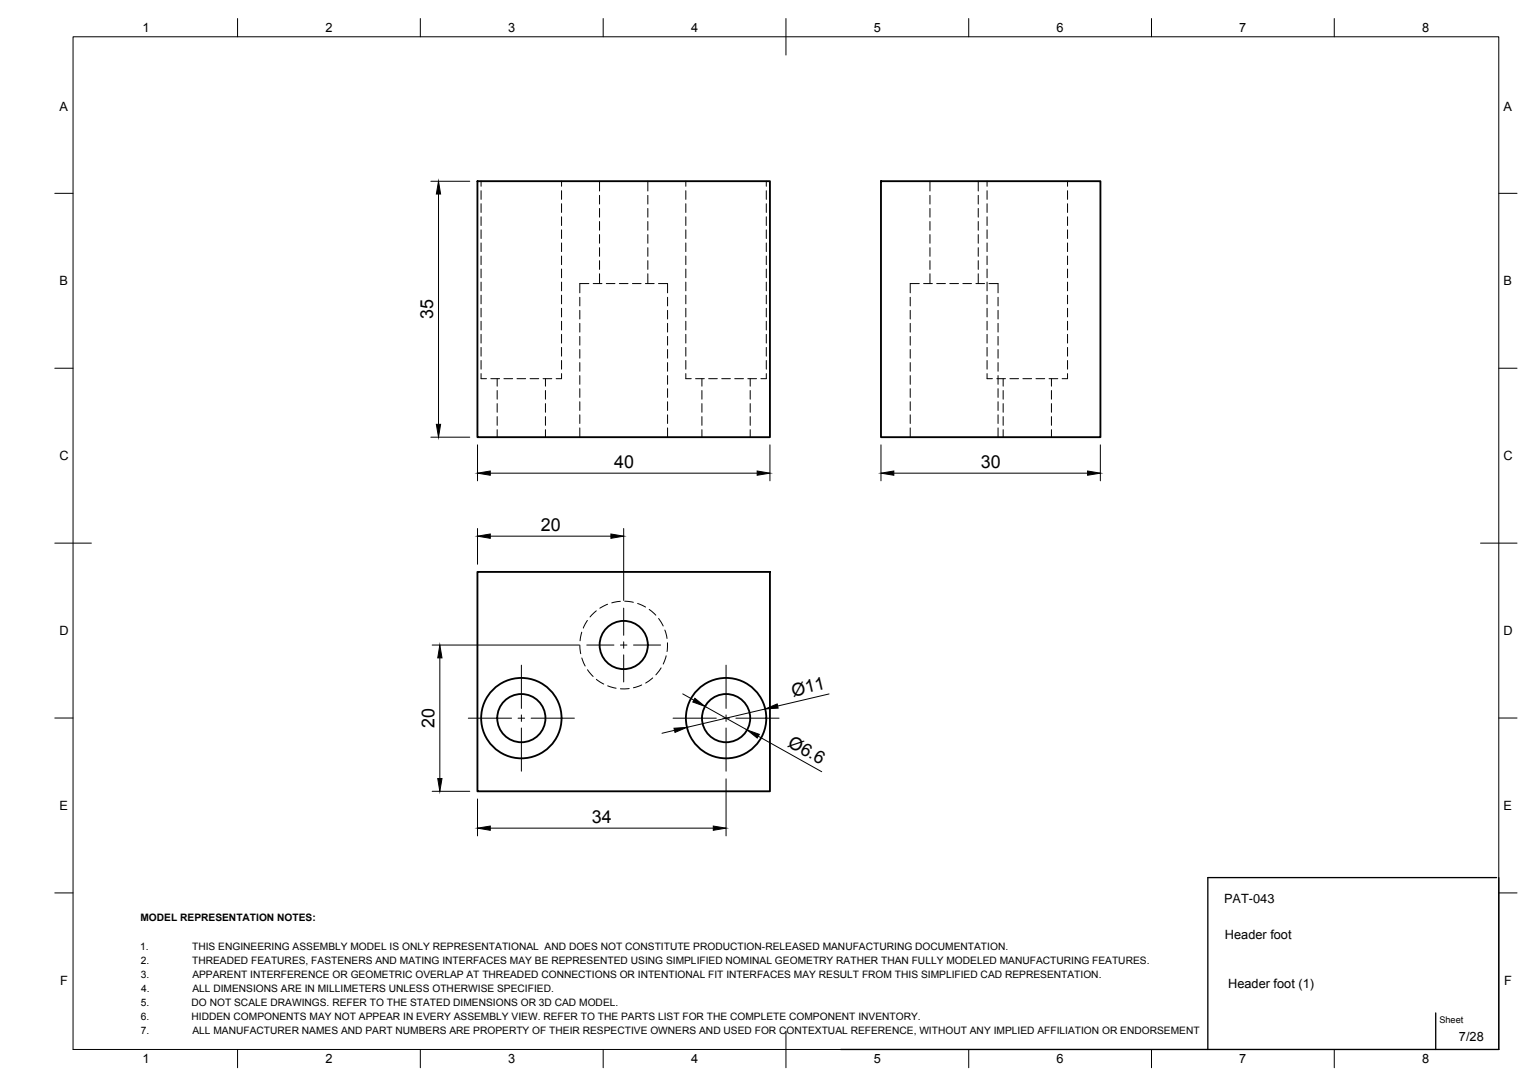
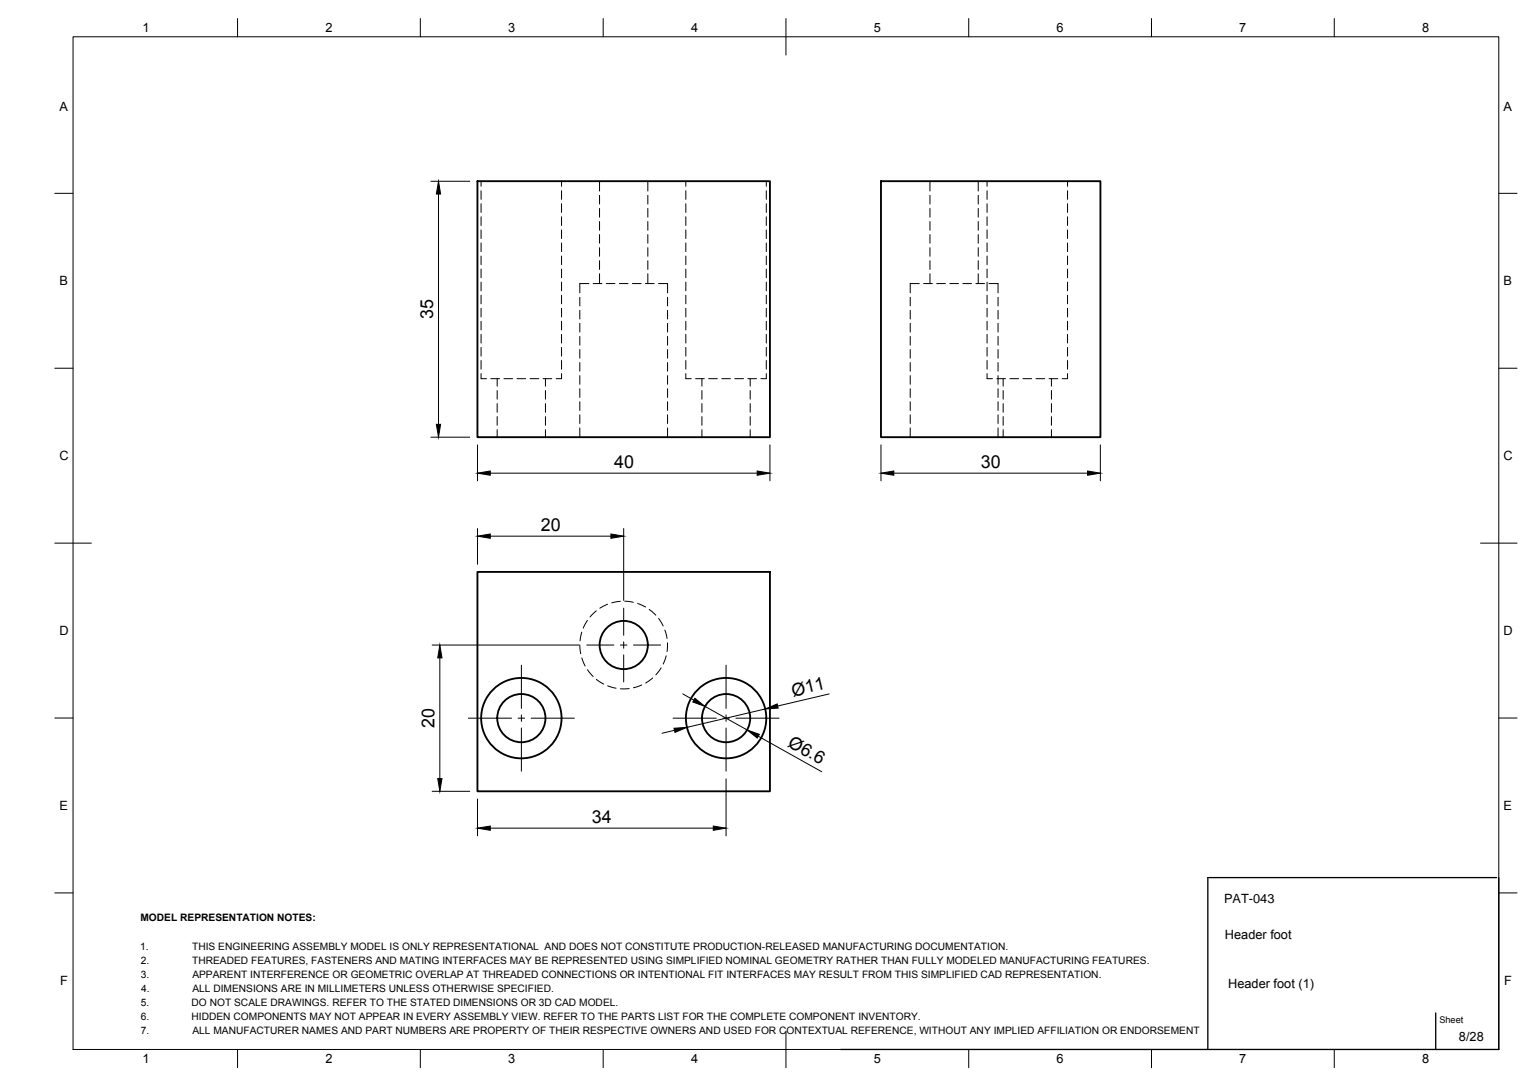
ISO-10303-21;
HEADER;
/* Generated by software containing ST-Developer
 * from STEP Tools, Inc. (www.steptools.com) 
 */

FILE_DESCRIPTION(
/* description */ ('Four-valve pipe header'),
/* implementation_level */ '2;1');

FILE_NAME(
/* name */ 'Header foot.step',
/* time_stamp */ '2026-10-29T16:56:19-07:00',
/* author */ (''),
/* organization */ (''),
/* preprocessor_version */ 'ST-DEVELOPER v20.2',
/* originating_system */ 'Autodesk Translation Framework v15.17.0.0',
/* authorisation */ '');

FILE_SCHEMA (('AUTOMOTIVE_DESIGN { 1 0 10303 214 3 1 1 }'));
ENDSEC;

DATA;
#10=MECHANICAL_DESIGN_GEOMETRIC_PRESENTATION_REPRESENTATION('',(#335),#10119);
#283=SHAPE_REPRESENTATION_RELATIONSHIP('SRR','None',#10244,#309);
#309=ADVANCED_BREP_SHAPE_REPRESENTATION('',(#361),#10093);
#335=STYLED_ITEM('',(#10463),#361);
#361=MANIFOLD_SOLID_BREP('Body1',#5581);
#437=FACE_BOUND('',#1153,.T.);
#438=FACE_BOUND('',#1157,.T.);
#439=FACE_BOUND('',#1161,.T.);
#440=FACE_BOUND('',#1168,.T.);
#441=FACE_BOUND('',#1169,.T.);
#442=FACE_BOUND('',#1170,.T.);
#443=FACE_BOUND('',#1172,.T.);
#444=FACE_BOUND('',#1173,.T.);
#445=FACE_BOUND('',#1174,.T.);
#570=PLANE('',#6036);
#571=PLANE('',#6043);
#572=PLANE('',#6050);
#573=PLANE('',#6054);
#574=PLANE('',#6055);
#575=PLANE('',#6056);
#576=PLANE('',#6057);
#577=PLANE('',#6058);
#578=PLANE('',#6059);
#808=FACE_OUTER_BOUND('',#1151,.T.);
#809=FACE_OUTER_BOUND('',#1152,.T.);
#810=FACE_OUTER_BOUND('',#1154,.T.);
#811=FACE_OUTER_BOUND('',#1155,.T.);
#812=FACE_OUTER_BOUND('',#1156,.T.);
#813=FACE_OUTER_BOUND('',#1158,.T.);
#814=FACE_OUTER_BOUND('',#1159,.T.);
#815=FACE_OUTER_BOUND('',#1160,.T.);
#816=FACE_OUTER_BOUND('',#1162,.T.);
#817=FACE_OUTER_BOUND('',#1163,.T.);
#818=FACE_OUTER_BOUND('',#1164,.T.);
#819=FACE_OUTER_BOUND('',#1165,.T.);
#820=FACE_OUTER_BOUND('',#1166,.T.);
#821=FACE_OUTER_BOUND('',#1167,.T.);
#822=FACE_OUTER_BOUND('',#1171,.T.);
#1151=EDGE_LOOP('',(#4045,#4046,#4047,#4048));
#1152=EDGE_LOOP('',(#4049));
#1153=EDGE_LOOP('',(#4050));
#1154=EDGE_LOOP('',(#4051,#4052,#4053,#4054));
#1155=EDGE_LOOP('',(#4055,#4056,#4057,#4058));
#1156=EDGE_LOOP('',(#4059));
#1157=EDGE_LOOP('',(#4060));
#1158=EDGE_LOOP('',(#4061,#4062,#4063,#4064));
#1159=EDGE_LOOP('',(#4065,#4066,#4067,#4068));
#1160=EDGE_LOOP('',(#4069));
#1161=EDGE_LOOP('',(#4070));
#1162=EDGE_LOOP('',(#4071,#4072,#4073,#4074));
#1163=EDGE_LOOP('',(#4075,#4076,#4077,#4078));
#1164=EDGE_LOOP('',(#4079,#4080,#4081,#4082));
#1165=EDGE_LOOP('',(#4083,#4084,#4085,#4086));
#1166=EDGE_LOOP('',(#4087,#4088,#4089,#4090));
#1167=EDGE_LOOP('',(#4091,#4092,#4093,#4094));
#1168=EDGE_LOOP('',(#4095));
#1169=EDGE_LOOP('',(#4096));
#1170=EDGE_LOOP('',(#4097));
#1171=EDGE_LOOP('',(#4098,#4099,#4100,#4101));
#1172=EDGE_LOOP('',(#4102));
#1173=EDGE_LOOP('',(#4103));
#1174=EDGE_LOOP('',(#4104));
#1588=LINE('',#8761,#2006);
#1589=LINE('',#8769,#2007);
#1590=LINE('',#8774,#2008);
#1591=LINE('',#8782,#2009);
#1592=LINE('',#8787,#2010);
#1593=LINE('',#8794,#2011);
#1594=LINE('',#8799,#2012);
#1595=LINE('',#8801,#2013);
#1596=LINE('',#8803,#2014);
#1597=LINE('',#8804,#2015);
#1598=LINE('',#8807,#2016);
#1599=LINE('',#8809,#2017);
#1600=LINE('',#8810,#2018);
#1601=LINE('',#8813,#2019);
#1602=LINE('',#8815,#2020);
#1603=LINE('',#8816,#2021);
#1604=LINE('',#8818,#2022);
#1605=LINE('',#8819,#2023);
#2006=VECTOR('',#6917,0.55);
#2007=VECTOR('',#6928,0.33);
#2008=VECTOR('',#6933,0.55);
#2009=VECTOR('',#6944,0.33);
#2010=VECTOR('',#6949,0.6);
#2011=VECTOR('',#6958,0.33);
#2012=VECTOR('',#6963,1.);
#2013=VECTOR('',#6964,1.);
#2014=VECTOR('',#6965,1.);
#2015=VECTOR('',#6966,1.);
#2016=VECTOR('',#6969,1.);
#2017=VECTOR('',#6970,1.);
#2018=VECTOR('',#6971,1.);
#2019=VECTOR('',#6974,1.);
#2020=VECTOR('',#6975,1.);
#2021=VECTOR('',#6976,1.);
#2022=VECTOR('',#6979,1.);
#2023=VECTOR('',#6980,1.);
#2396=CIRCLE('',#6034,0.55);
#2397=CIRCLE('',#6035,0.55);
#2398=CIRCLE('',#6037,0.33);
#2399=CIRCLE('',#6039,0.33);
#2400=CIRCLE('',#6041,0.55);
#2401=CIRCLE('',#6042,0.55);
#2402=CIRCLE('',#6044,0.33);
#2403=CIRCLE('',#6046,0.33);
#2404=CIRCLE('',#6048,0.6);
#2405=CIRCLE('',#6049,0.6);
#2406=CIRCLE('',#6051,0.33);
#2407=CIRCLE('',#6053,0.33);
#2676=VERTEX_POINT('',#8758);
#2677=VERTEX_POINT('',#8760);
#2678=VERTEX_POINT('',#8764);
#2679=VERTEX_POINT('',#8767);
#2680=VERTEX_POINT('',#8771);
#2681=VERTEX_POINT('',#8773);
#2682=VERTEX_POINT('',#8777);
#2683=VERTEX_POINT('',#8780);
#2684=VERTEX_POINT('',#8784);
#2685=VERTEX_POINT('',#8786);
#2686=VERTEX_POINT('',#8790);
#2687=VERTEX_POINT('',#8793);
#2688=VERTEX_POINT('',#8797);
#2689=VERTEX_POINT('',#8798);
#2690=VERTEX_POINT('',#8800);
#2691=VERTEX_POINT('',#8802);
#2692=VERTEX_POINT('',#8806);
#2693=VERTEX_POINT('',#8808);
#2694=VERTEX_POINT('',#8812);
#2695=VERTEX_POINT('',#8814);
#3189=EDGE_CURVE('',#2676,#2676,#2396,.T.);
#3190=EDGE_CURVE('',#2676,#2677,#1588,.T.);
#3191=EDGE_CURVE('',#2677,#2677,#2397,.T.);
#3192=EDGE_CURVE('',#2678,#2678,#2398,.T.);
#3193=EDGE_CURVE('',#2679,#2679,#2399,.T.);
#3194=EDGE_CURVE('',#2679,#2678,#1589,.T.);
#3195=EDGE_CURVE('',#2680,#2680,#2400,.T.);
#3196=EDGE_CURVE('',#2680,#2681,#1590,.T.);
#3197=EDGE_CURVE('',#2681,#2681,#2401,.T.);
#3198=EDGE_CURVE('',#2682,#2682,#2402,.T.);
#3199=EDGE_CURVE('',#2683,#2683,#2403,.T.);
#3200=EDGE_CURVE('',#2683,#2682,#1591,.T.);
#3201=EDGE_CURVE('',#2684,#2684,#2404,.T.);
#3202=EDGE_CURVE('',#2684,#2685,#1592,.T.);
#3203=EDGE_CURVE('',#2685,#2685,#2405,.T.);
#3204=EDGE_CURVE('',#2686,#2686,#2406,.T.);
#3205=EDGE_CURVE('',#2686,#2687,#1593,.T.);
#3206=EDGE_CURVE('',#2687,#2687,#2407,.T.);
#3207=EDGE_CURVE('',#2688,#2689,#1594,.T.);
#3208=EDGE_CURVE('',#2689,#2690,#1595,.T.);
#3209=EDGE_CURVE('',#2691,#2690,#1596,.T.);
#3210=EDGE_CURVE('',#2688,#2691,#1597,.T.);
#3211=EDGE_CURVE('',#2692,#2688,#1598,.T.);
#3212=EDGE_CURVE('',#2693,#2691,#1599,.T.);
#3213=EDGE_CURVE('',#2692,#2693,#1600,.T.);
#3214=EDGE_CURVE('',#2694,#2692,#1601,.T.);
#3215=EDGE_CURVE('',#2695,#2693,#1602,.T.);
#3216=EDGE_CURVE('',#2694,#2695,#1603,.T.);
#3217=EDGE_CURVE('',#2689,#2694,#1604,.T.);
#3218=EDGE_CURVE('',#2690,#2695,#1605,.T.);
#4045=ORIENTED_EDGE('',*,*,#3189,.F.);
#4046=ORIENTED_EDGE('',*,*,#3190,.T.);
#4047=ORIENTED_EDGE('',*,*,#3191,.F.);
#4048=ORIENTED_EDGE('',*,*,#3190,.F.);
#4049=ORIENTED_EDGE('',*,*,#3189,.T.);
#4050=ORIENTED_EDGE('',*,*,#3192,.F.);
#4051=ORIENTED_EDGE('',*,*,#3193,.F.);
#4052=ORIENTED_EDGE('',*,*,#3194,.T.);
#4053=ORIENTED_EDGE('',*,*,#3192,.T.);
#4054=ORIENTED_EDGE('',*,*,#3194,.F.);
#4055=ORIENTED_EDGE('',*,*,#3195,.F.);
#4056=ORIENTED_EDGE('',*,*,#3196,.T.);
#4057=ORIENTED_EDGE('',*,*,#3197,.F.);
#4058=ORIENTED_EDGE('',*,*,#3196,.F.);
#4059=ORIENTED_EDGE('',*,*,#3195,.T.);
#4060=ORIENTED_EDGE('',*,*,#3198,.F.);
#4061=ORIENTED_EDGE('',*,*,#3199,.F.);
#4062=ORIENTED_EDGE('',*,*,#3200,.T.);
#4063=ORIENTED_EDGE('',*,*,#3198,.T.);
#4064=ORIENTED_EDGE('',*,*,#3200,.F.);
#4065=ORIENTED_EDGE('',*,*,#3201,.F.);
#4066=ORIENTED_EDGE('',*,*,#3202,.T.);
#4067=ORIENTED_EDGE('',*,*,#3203,.T.);
#4068=ORIENTED_EDGE('',*,*,#3202,.F.);
#4069=ORIENTED_EDGE('',*,*,#3203,.F.);
#4070=ORIENTED_EDGE('',*,*,#3204,.F.);
#4071=ORIENTED_EDGE('',*,*,#3204,.T.);
#4072=ORIENTED_EDGE('',*,*,#3205,.T.);
#4073=ORIENTED_EDGE('',*,*,#3206,.F.);
#4074=ORIENTED_EDGE('',*,*,#3205,.F.);
#4075=ORIENTED_EDGE('',*,*,#3207,.T.);
#4076=ORIENTED_EDGE('',*,*,#3208,.T.);
#4077=ORIENTED_EDGE('',*,*,#3209,.F.);
#4078=ORIENTED_EDGE('',*,*,#3210,.F.);
#4079=ORIENTED_EDGE('',*,*,#3211,.T.);
#4080=ORIENTED_EDGE('',*,*,#3210,.T.);
#4081=ORIENTED_EDGE('',*,*,#3212,.F.);
#4082=ORIENTED_EDGE('',*,*,#3213,.F.);
#4083=ORIENTED_EDGE('',*,*,#3214,.T.);
#4084=ORIENTED_EDGE('',*,*,#3213,.T.);
#4085=ORIENTED_EDGE('',*,*,#3215,.F.);
#4086=ORIENTED_EDGE('',*,*,#3216,.F.);
#4087=ORIENTED_EDGE('',*,*,#3217,.T.);
#4088=ORIENTED_EDGE('',*,*,#3216,.T.);
#4089=ORIENTED_EDGE('',*,*,#3218,.F.);
#4090=ORIENTED_EDGE('',*,*,#3208,.F.);
#4091=ORIENTED_EDGE('',*,*,#3218,.T.);
#4092=ORIENTED_EDGE('',*,*,#3215,.T.);
#4093=ORIENTED_EDGE('',*,*,#3212,.T.);
#4094=ORIENTED_EDGE('',*,*,#3209,.T.);
#4095=ORIENTED_EDGE('',*,*,#3191,.T.);
#4096=ORIENTED_EDGE('',*,*,#3197,.T.);
#4097=ORIENTED_EDGE('',*,*,#3206,.T.);
#4098=ORIENTED_EDGE('',*,*,#3217,.F.);
#4099=ORIENTED_EDGE('',*,*,#3207,.F.);
#4100=ORIENTED_EDGE('',*,*,#3211,.F.);
#4101=ORIENTED_EDGE('',*,*,#3214,.F.);
#4102=ORIENTED_EDGE('',*,*,#3193,.T.);
#4103=ORIENTED_EDGE('',*,*,#3199,.T.);
#4104=ORIENTED_EDGE('',*,*,#3201,.T.);
#5175=CYLINDRICAL_SURFACE('',#6033,0.55);
#5176=CYLINDRICAL_SURFACE('',#6038,0.33);
#5177=CYLINDRICAL_SURFACE('',#6040,0.55);
#5178=CYLINDRICAL_SURFACE('',#6045,0.33);
#5179=CYLINDRICAL_SURFACE('',#6047,0.6);
#5180=CYLINDRICAL_SURFACE('',#6052,0.33);
#5308=ADVANCED_FACE('',(#808),#5175,.F.);
#5309=ADVANCED_FACE('',(#809,#437),#570,.T.);
#5310=ADVANCED_FACE('',(#810),#5176,.F.);
#5311=ADVANCED_FACE('',(#811),#5177,.F.);
#5312=ADVANCED_FACE('',(#812,#438),#571,.T.);
#5313=ADVANCED_FACE('',(#813),#5178,.F.);
#5314=ADVANCED_FACE('',(#814),#5179,.F.);
#5315=ADVANCED_FACE('',(#815,#439),#572,.F.);
#5316=ADVANCED_FACE('',(#816),#5180,.F.);
#5317=ADVANCED_FACE('',(#817),#573,.T.);
#5318=ADVANCED_FACE('',(#818),#574,.T.);
#5319=ADVANCED_FACE('',(#819),#575,.T.);
#5320=ADVANCED_FACE('',(#820),#576,.T.);
#5321=ADVANCED_FACE('',(#821,#440,#441,#442),#577,.T.);
#5322=ADVANCED_FACE('',(#822,#443,#444,#445),#578,.F.);
#5581=CLOSED_SHELL('',(#5308,#5309,#5310,#5311,#5312,#5313,#5314,#5315,
#5316,#5317,#5318,#5319,#5320,#5321,#5322));
#6032=AXIS2_PLACEMENT_3D('',#8756,#6911,#6912);
#6033=AXIS2_PLACEMENT_3D('',#8757,#6913,#6914);
#6034=AXIS2_PLACEMENT_3D('',#8759,#6915,#6916);
#6035=AXIS2_PLACEMENT_3D('',#8762,#6918,#6919);
#6036=AXIS2_PLACEMENT_3D('',#8763,#6920,#6921);
#6037=AXIS2_PLACEMENT_3D('',#8765,#6922,#6923);
#6038=AXIS2_PLACEMENT_3D('',#8766,#6924,#6925);
#6039=AXIS2_PLACEMENT_3D('',#8768,#6926,#6927);
#6040=AXIS2_PLACEMENT_3D('',#8770,#6929,#6930);
#6041=AXIS2_PLACEMENT_3D('',#8772,#6931,#6932);
#6042=AXIS2_PLACEMENT_3D('',#8775,#6934,#6935);
#6043=AXIS2_PLACEMENT_3D('',#8776,#6936,#6937);
#6044=AXIS2_PLACEMENT_3D('',#8778,#6938,#6939);
#6045=AXIS2_PLACEMENT_3D('',#8779,#6940,#6941);
#6046=AXIS2_PLACEMENT_3D('',#8781,#6942,#6943);
#6047=AXIS2_PLACEMENT_3D('',#8783,#6945,#6946);
#6048=AXIS2_PLACEMENT_3D('',#8785,#6947,#6948);
#6049=AXIS2_PLACEMENT_3D('',#8788,#6950,#6951);
#6050=AXIS2_PLACEMENT_3D('',#8789,#6952,#6953);
#6051=AXIS2_PLACEMENT_3D('',#8791,#6954,#6955);
#6052=AXIS2_PLACEMENT_3D('',#8792,#6956,#6957);
#6053=AXIS2_PLACEMENT_3D('',#8795,#6959,#6960);
#6054=AXIS2_PLACEMENT_3D('',#8796,#6961,#6962);
#6055=AXIS2_PLACEMENT_3D('',#8805,#6967,#6968);
#6056=AXIS2_PLACEMENT_3D('',#8811,#6972,#6973);
#6057=AXIS2_PLACEMENT_3D('',#8817,#6977,#6978);
#6058=AXIS2_PLACEMENT_3D('',#8820,#6981,#6982);
#6059=AXIS2_PLACEMENT_3D('',#8821,#6983,#6984);
#6911=DIRECTION('axis',(0.,0.,1.));
#6912=DIRECTION('refdir',(1.,0.,0.));
#6913=DIRECTION('center_axis',(0.,0.,1.));
#6914=DIRECTION('ref_axis',(1.,0.,0.));
#6915=DIRECTION('center_axis',(0.,0.,1.));
#6916=DIRECTION('ref_axis',(1.,0.,0.));
#6917=DIRECTION('',(0.,0.,1.));
#6918=DIRECTION('center_axis',(0.,0.,-1.));
#6919=DIRECTION('ref_axis',(1.,0.,0.));
#6920=DIRECTION('center_axis',(0.,0.,1.));
#6921=DIRECTION('ref_axis',(1.,0.,0.));
#6922=DIRECTION('center_axis',(0.,0.,1.));
#6923=DIRECTION('ref_axis',(1.,0.,0.));
#6924=DIRECTION('center_axis',(0.,0.,1.));
#6925=DIRECTION('ref_axis',(1.,0.,0.));
#6926=DIRECTION('center_axis',(0.,0.,1.));
#6927=DIRECTION('ref_axis',(1.,0.,0.));
#6928=DIRECTION('',(0.,0.,1.));
#6929=DIRECTION('center_axis',(0.,0.,1.));
#6930=DIRECTION('ref_axis',(1.,0.,0.));
#6931=DIRECTION('center_axis',(0.,0.,1.));
#6932=DIRECTION('ref_axis',(1.,0.,0.));
#6933=DIRECTION('',(0.,0.,1.));
#6934=DIRECTION('center_axis',(0.,0.,-1.));
#6935=DIRECTION('ref_axis',(1.,0.,0.));
#6936=DIRECTION('center_axis',(0.,0.,1.));
#6937=DIRECTION('ref_axis',(1.,0.,0.));
#6938=DIRECTION('center_axis',(0.,0.,1.));
#6939=DIRECTION('ref_axis',(1.,0.,0.));
#6940=DIRECTION('center_axis',(0.,0.,1.));
#6941=DIRECTION('ref_axis',(1.,0.,0.));
#6942=DIRECTION('center_axis',(0.,0.,1.));
#6943=DIRECTION('ref_axis',(1.,0.,0.));
#6944=DIRECTION('',(0.,0.,1.));
#6945=DIRECTION('center_axis',(0.,0.,1.));
#6946=DIRECTION('ref_axis',(1.,0.,0.));
#6947=DIRECTION('center_axis',(0.,0.,1.));
#6948=DIRECTION('ref_axis',(1.,0.,0.));
#6949=DIRECTION('',(0.,0.,1.));
#6950=DIRECTION('center_axis',(0.,0.,1.));
#6951=DIRECTION('ref_axis',(1.,0.,0.));
#6952=DIRECTION('center_axis',(0.,0.,1.));
#6953=DIRECTION('ref_axis',(1.,0.,0.));
#6954=DIRECTION('center_axis',(0.,0.,-1.));
#6955=DIRECTION('ref_axis',(1.,0.,0.));
#6956=DIRECTION('center_axis',(0.,0.,1.));
#6957=DIRECTION('ref_axis',(1.,0.,0.));
#6958=DIRECTION('',(0.,0.,1.));
#6959=DIRECTION('center_axis',(0.,0.,-1.));
#6960=DIRECTION('ref_axis',(1.,0.,0.));
#6961=DIRECTION('center_axis',(0.,1.,0.));
#6962=DIRECTION('ref_axis',(-1.,0.,0.));
#6963=DIRECTION('',(-1.,0.,0.));
#6964=DIRECTION('',(0.,0.,1.));
#6965=DIRECTION('',(-1.,0.,0.));
#6966=DIRECTION('',(0.,0.,1.));
#6967=DIRECTION('center_axis',(1.,0.,0.));
#6968=DIRECTION('ref_axis',(0.,1.,0.));
#6969=DIRECTION('',(0.,1.,0.));
#6970=DIRECTION('',(0.,1.,0.));
#6971=DIRECTION('',(0.,0.,1.));
#6972=DIRECTION('center_axis',(0.,-1.,0.));
#6973=DIRECTION('ref_axis',(1.,0.,0.));
#6974=DIRECTION('',(1.,0.,0.));
#6975=DIRECTION('',(1.,0.,0.));
#6976=DIRECTION('',(0.,0.,1.));
#6977=DIRECTION('center_axis',(-1.,0.,0.));
#6978=DIRECTION('ref_axis',(0.,-1.,0.));
#6979=DIRECTION('',(0.,-1.,0.));
#6980=DIRECTION('',(0.,-1.,0.));
#6981=DIRECTION('center_axis',(0.,0.,1.));
#6982=DIRECTION('ref_axis',(1.,0.,0.));
#6983=DIRECTION('center_axis',(0.,0.,1.));
#6984=DIRECTION('ref_axis',(1.,0.,0.));
#8756=CARTESIAN_POINT('',(0.,0.,0.));
#8757=CARTESIAN_POINT('Origin',(-1.1,10.,0.8));
#8758=CARTESIAN_POINT('',(-1.65,10.,0.8));
#8759=CARTESIAN_POINT('Origin',(-1.1,10.,0.8));
#8760=CARTESIAN_POINT('',(-1.65,10.,3.5));
#8761=CARTESIAN_POINT('',(-1.65,10.,0.8));
#8762=CARTESIAN_POINT('Origin',(-1.1,10.,3.5));
#8763=CARTESIAN_POINT('Origin',(-1.1,10.,0.8));
#8764=CARTESIAN_POINT('',(-1.43,10.,0.8));
#8765=CARTESIAN_POINT('Origin',(-1.1,10.,0.8));
#8766=CARTESIAN_POINT('Origin',(-1.1,10.,-0.1));
#8767=CARTESIAN_POINT('',(-1.43,10.,0.));
#8768=CARTESIAN_POINT('Origin',(-1.1,10.,0.));
#8769=CARTESIAN_POINT('',(-1.43,10.,-0.1));
#8770=CARTESIAN_POINT('Origin',(-3.9,10.,0.8));
#8771=CARTESIAN_POINT('',(-4.45,10.,0.8));
#8772=CARTESIAN_POINT('Origin',(-3.9,10.,0.8));
#8773=CARTESIAN_POINT('',(-4.45,10.,3.5));
#8774=CARTESIAN_POINT('',(-4.45,10.,0.8));
#8775=CARTESIAN_POINT('Origin',(-3.9,10.,3.5));
#8776=CARTESIAN_POINT('Origin',(-3.9,10.,0.8));
#8777=CARTESIAN_POINT('',(-4.23,10.,0.8));
#8778=CARTESIAN_POINT('Origin',(-3.9,10.,0.8));
#8779=CARTESIAN_POINT('Origin',(-3.9,10.,-0.1));
#8780=CARTESIAN_POINT('',(-4.23,10.,0.));
#8781=CARTESIAN_POINT('Origin',(-3.9,10.,0.));
#8782=CARTESIAN_POINT('',(-4.23,10.,-0.1));
#8783=CARTESIAN_POINT('Origin',(-2.5,9.,-0.1));
#8784=CARTESIAN_POINT('',(-3.1,9.,0.));
#8785=CARTESIAN_POINT('Origin',(-2.5,9.,0.));
#8786=CARTESIAN_POINT('',(-3.1,9.,2.1));
#8787=CARTESIAN_POINT('',(-3.1,9.,-0.1));
#8788=CARTESIAN_POINT('Origin',(-2.5,9.,2.1));
#8789=CARTESIAN_POINT('Origin',(-2.5,9.,2.1));
#8790=CARTESIAN_POINT('',(-2.83,9.,2.1));
#8791=CARTESIAN_POINT('Origin',(-2.5,9.,2.1));
#8792=CARTESIAN_POINT('Origin',(-2.5,9.,-0.1));
#8793=CARTESIAN_POINT('',(-2.83,9.,3.5));
#8794=CARTESIAN_POINT('',(-2.83,9.,-0.1));
#8795=CARTESIAN_POINT('Origin',(-2.5,9.,3.5));
#8796=CARTESIAN_POINT('Origin',(-0.5,11.,0.));
#8797=CARTESIAN_POINT('',(-0.5,11.,0.));
#8798=CARTESIAN_POINT('',(-4.5,11.,0.));
#8799=CARTESIAN_POINT('',(-0.5,11.,0.));
#8800=CARTESIAN_POINT('',(-4.5,11.,3.5));
#8801=CARTESIAN_POINT('',(-4.5,11.,0.));
#8802=CARTESIAN_POINT('',(-0.5,11.,3.5));
#8803=CARTESIAN_POINT('',(-0.5,11.,3.5));
#8804=CARTESIAN_POINT('',(-0.5,11.,0.));
#8805=CARTESIAN_POINT('Origin',(-0.5,8.,0.));
#8806=CARTESIAN_POINT('',(-0.5,8.,0.));
#8807=CARTESIAN_POINT('',(-0.5,8.,0.));
#8808=CARTESIAN_POINT('',(-0.5,8.,3.5));
#8809=CARTESIAN_POINT('',(-0.5,8.,3.5));
#8810=CARTESIAN_POINT('',(-0.5,8.,0.));
#8811=CARTESIAN_POINT('Origin',(-4.5,8.,0.));
#8812=CARTESIAN_POINT('',(-4.5,8.,0.));
#8813=CARTESIAN_POINT('',(-4.5,8.,0.));
#8814=CARTESIAN_POINT('',(-4.5,8.,3.5));
#8815=CARTESIAN_POINT('',(-4.5,8.,3.5));
#8816=CARTESIAN_POINT('',(-4.5,8.,0.));
#8817=CARTESIAN_POINT('Origin',(-4.5,11.,0.));
#8818=CARTESIAN_POINT('',(-4.5,11.,0.));
#8819=CARTESIAN_POINT('',(-4.5,11.,3.5));
#8820=CARTESIAN_POINT('Origin',(-2.5,9.5,3.5));
#8821=CARTESIAN_POINT('Origin',(-2.5,9.5,0.));
#10062=UNCERTAINTY_MEASURE_WITH_UNIT(LENGTH_MEASURE(0.001),#10120,
'DISTANCE_ACCURACY_VALUE',
'Maximum model space distance between geometric entities at asserted c
onnectivities');
#10088=UNCERTAINTY_MEASURE_WITH_UNIT(LENGTH_MEASURE(0.001),#10120,
'DISTANCE_ACCURACY_VALUE',
'Maximum model space distance between geometric entities at asserted c
onnectivities');
#10093=(
GEOMETRIC_REPRESENTATION_CONTEXT(3)
GLOBAL_UNCERTAINTY_ASSIGNED_CONTEXT((#10062))
GLOBAL_UNIT_ASSIGNED_CONTEXT((#10120,#10122,#10123))
REPRESENTATION_CONTEXT('','3D')
);
#10119=(
GEOMETRIC_REPRESENTATION_CONTEXT(3)
GLOBAL_UNCERTAINTY_ASSIGNED_CONTEXT((#10088))
GLOBAL_UNIT_ASSIGNED_CONTEXT((#10120,#10122,#10123))
REPRESENTATION_CONTEXT('','3D')
);
#10120=(
LENGTH_UNIT()
NAMED_UNIT(*)
SI_UNIT(.CENTI.,.METRE.)
);
#10122=(
NAMED_UNIT(*)
PLANE_ANGLE_UNIT()
SI_UNIT($,.RADIAN.)
);
#10123=(
NAMED_UNIT(*)
SI_UNIT($,.STERADIAN.)
SOLID_ANGLE_UNIT()
);
#10128=SHAPE_DEFINITION_REPRESENTATION(#10158,#10244);
#10158=PRODUCT_DEFINITION_SHAPE('',$,#10275);
#10244=SHAPE_REPRESENTATION('',(#6032),#10093);
#10270=PRODUCT_DEFINITION_CONTEXT('part definition',#10362,'design');
#10275=PRODUCT_DEFINITION('Header foot','Header foot',#10305,#10270);
#10305=PRODUCT_DEFINITION_FORMATION('',$,#10368);
#10362=APPLICATION_CONTEXT(
'Core Data for Automotive Mechanical Design Process');
#10363=PRODUCT_CONTEXT('part definition',#10362,'mechanical');
#10368=PRODUCT('Header foot','Header foot','Header foot',(#10363));
#10457=COLOUR_RGB('Sky Blue',0.24,0.69,0.87);
#10458=FILL_AREA_STYLE_COLOUR('',#10457);
#10459=FILL_AREA_STYLE('',(#10458));
#10460=SURFACE_STYLE_FILL_AREA(#10459);
#10461=SURFACE_SIDE_STYLE('',(#10460));
#10462=SURFACE_STYLE_USAGE(.BOTH.,#10461);
#10463=PRESENTATION_STYLE_ASSIGNMENT((#10462));
ENDSEC;
END-ISO-10303-21;
